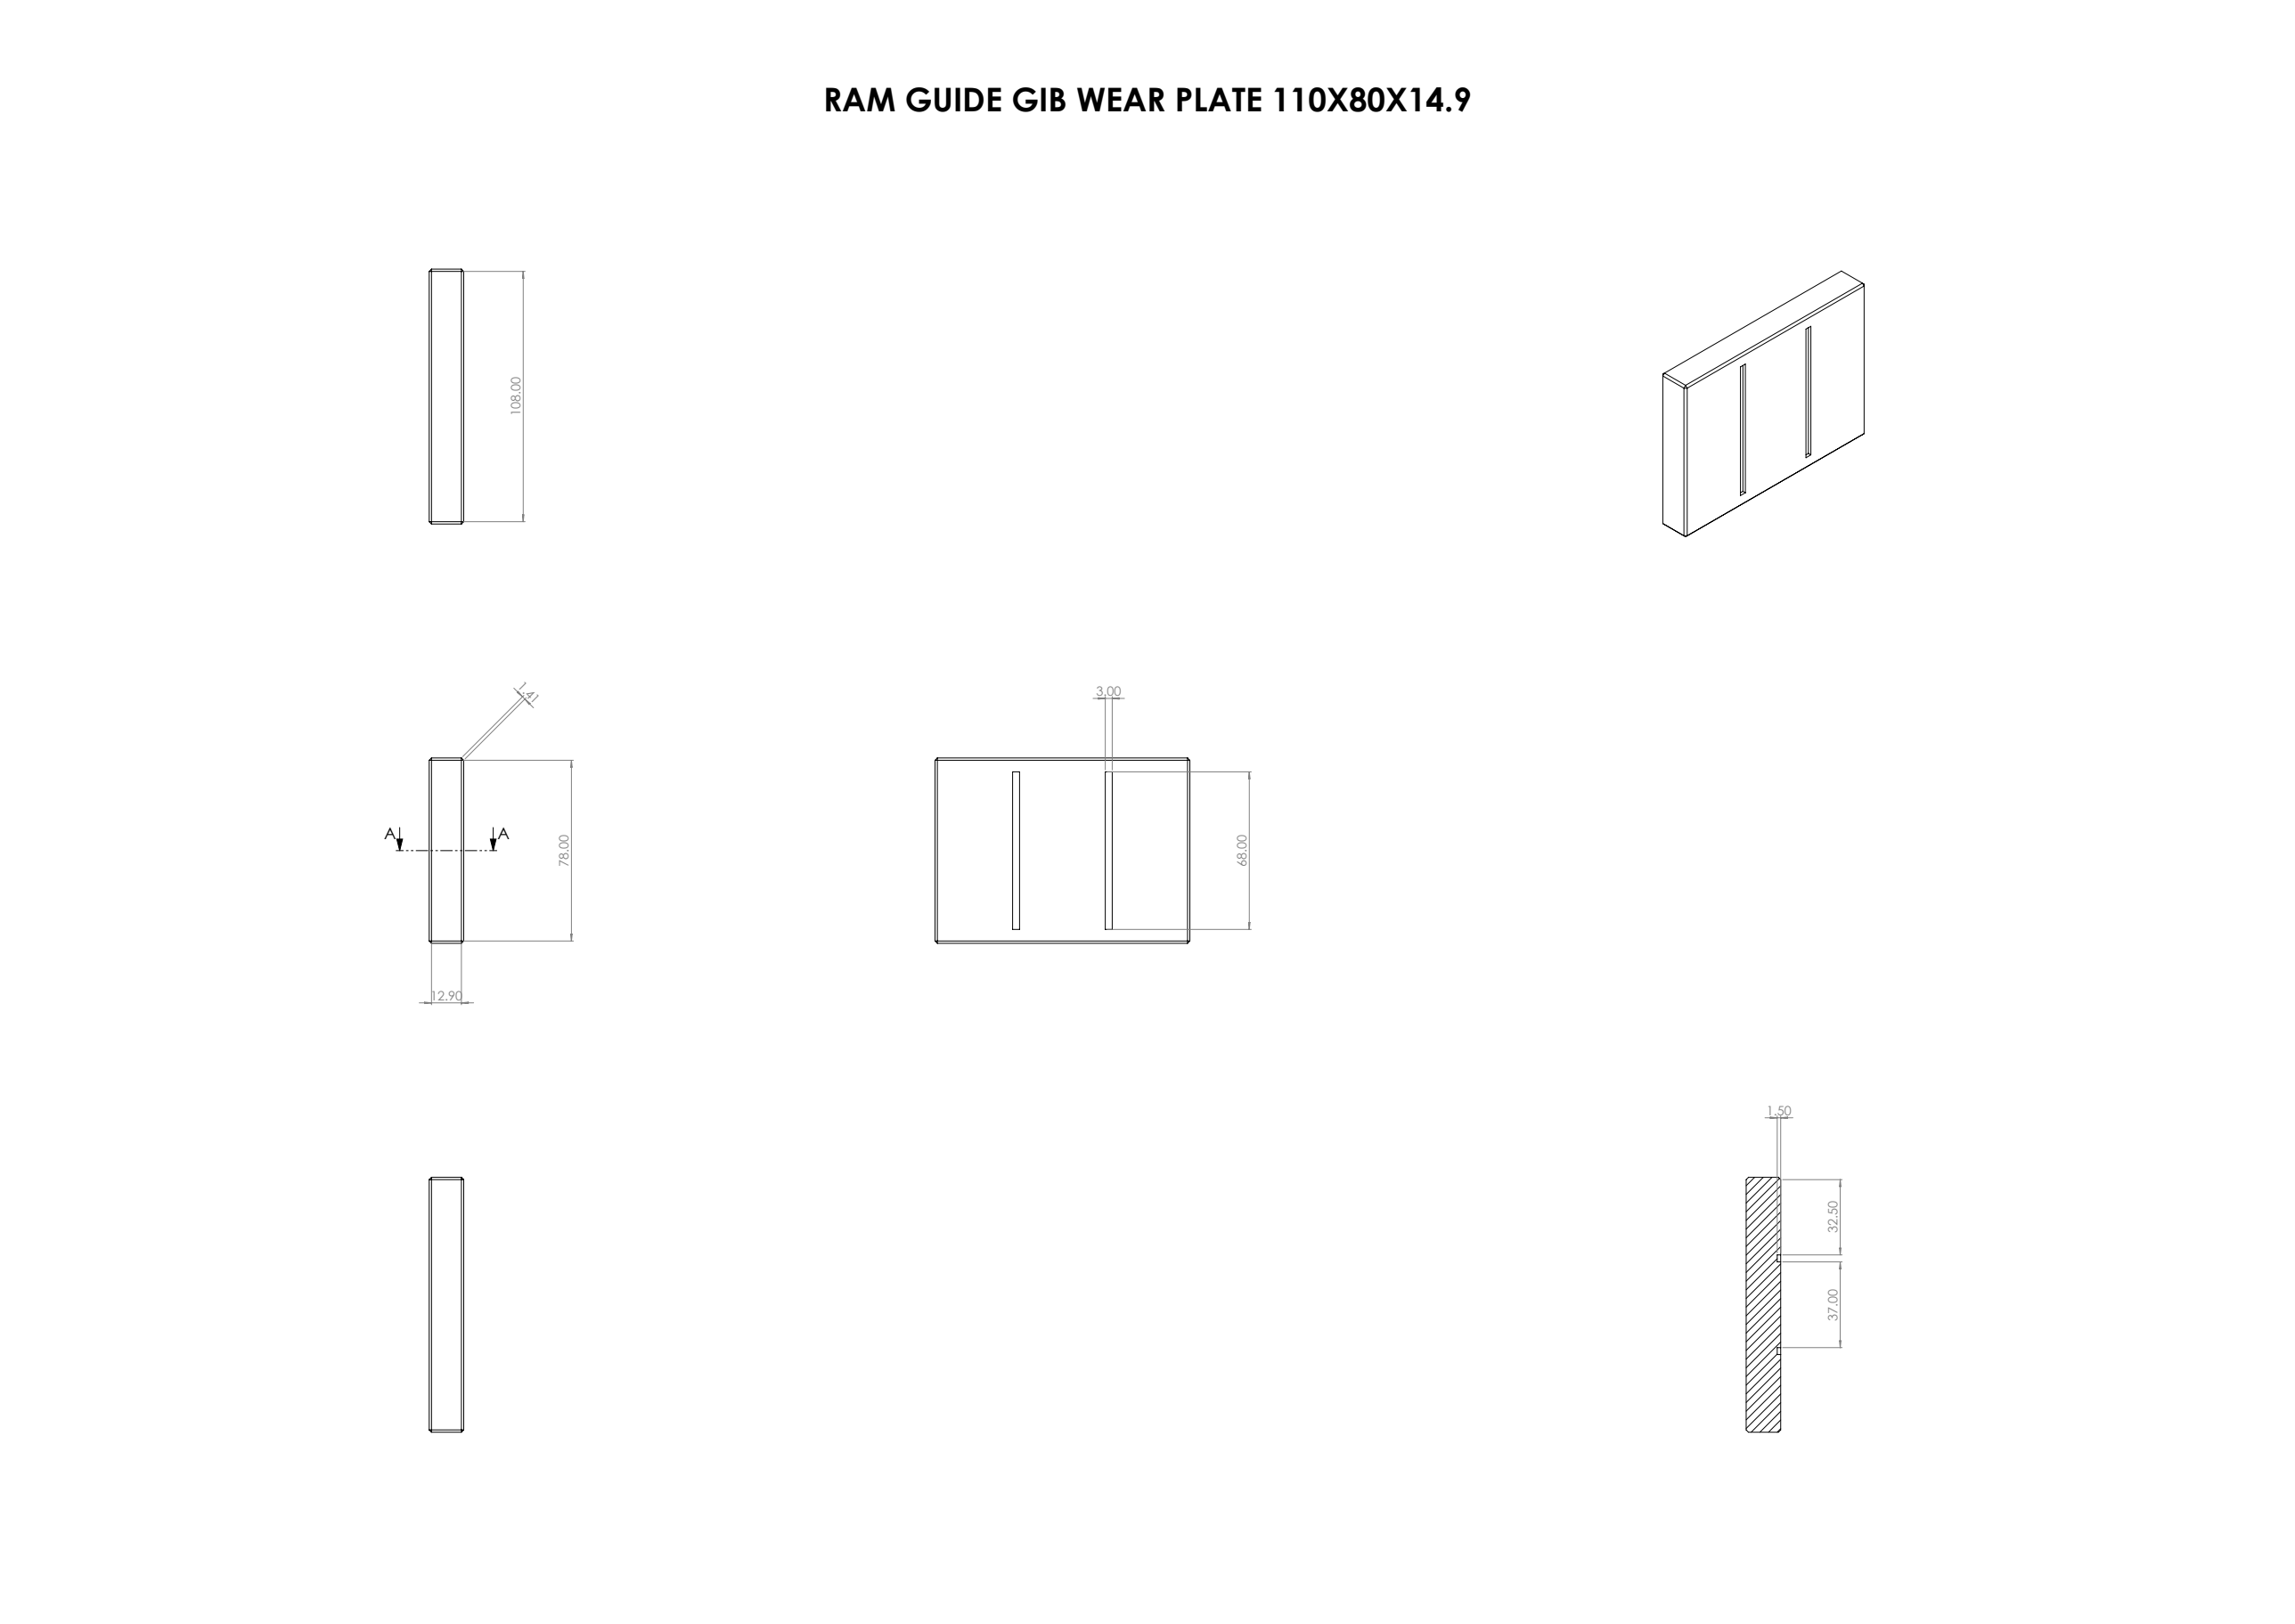
ISO-10303-21;
HEADER;
/* Generated by software containing ST-Developer
 * from STEP Tools, Inc. (www.steptools.com) 
 */

FILE_DESCRIPTION(
/* description */ (''),
/* implementation_level */ '2;1');

FILE_NAME(
/* name */ '10_Ram_Guide_Gib_Wear_Plate_110x80x14.9.step',
/* time_stamp */ '2026-10-19T23:58:09-07:00',
/* author */ (''),
/* organization */ (''),
/* preprocessor_version */ 'ST-DEVELOPER v20.2',
/* originating_system */ 'Autodesk Translation Framework v15.15.0.0',
/* authorisation */ '');

FILE_SCHEMA (('AP203_CONFIGURATION_CONTROLLED_3D_DESIGN_OF_MECHANICAL_PARTS_AND_ASSEMBLIES_MIM_LF { 1 0 10303 203 3 1 4 }',
'AUTOMOTIVE_DESIGN { 1 0 10303 214 3 1 1 }','INTEGRATED_CNC_SCHEMA','MODEL_BASED_INTEGRATED_MANUFACTURING_SCHEMA',
'PROCESS_PLANNING_SCHEMA','AP242_MANAGED_MODEL_BASED_3D_ENGINEERING_MIM_LF { 1 0 10303 442 3 1 4 }'));
ENDSEC;

DATA;
#10=MECHANICAL_DESIGN_GEOMETRIC_PRESENTATION_REPRESENTATION('',(#413),#70757);
#383=SHAPE_REPRESENTATION_RELATIONSHIP('SRR','None',#70824,#398);
#398=ADVANCED_BREP_SHAPE_REPRESENTATION('',(#473),#70748);
#413=STYLED_ITEM('',(#71040),#473);
#473=MANIFOLD_SOLID_BREP('Gib',#26878);
#862=FACE_BOUND('',#4417,.T.);
#863=FACE_BOUND('',#4418,.T.);
#1799=PLANE('',#27511);
#1800=PLANE('',#27512);
#1801=PLANE('',#27513);
#1802=PLANE('',#27514);
#1803=PLANE('',#27515);
#1804=PLANE('',#27516);
#1805=PLANE('',#27517);
#1806=PLANE('',#27518);
#1807=PLANE('',#27519);
#1808=PLANE('',#27520);
#1809=PLANE('',#27521);
#1810=PLANE('',#27522);
#1811=PLANE('',#27523);
#1812=PLANE('',#27524);
#1813=PLANE('',#27525);
#1814=PLANE('',#27526);
#1815=PLANE('',#27527);
#1816=PLANE('',#27528);
#1817=PLANE('',#27529);
#1818=PLANE('',#27530);
#1819=PLANE('',#27531);
#1820=PLANE('',#27532);
#1821=PLANE('',#27533);
#1822=PLANE('',#27534);
#1823=PLANE('',#27535);
#1824=PLANE('',#27536);
#1825=PLANE('',#27537);
#1826=PLANE('',#27538);
#1827=PLANE('',#27539);
#1828=PLANE('',#27540);
#1829=PLANE('',#27541);
#1830=PLANE('',#27542);
#1831=PLANE('',#27543);
#1832=PLANE('',#27544);
#1833=PLANE('',#27545);
#1834=PLANE('',#27546);
#2876=FACE_OUTER_BOUND('',#4382,.T.);
#2877=FACE_OUTER_BOUND('',#4383,.T.);
#2878=FACE_OUTER_BOUND('',#4384,.T.);
#2879=FACE_OUTER_BOUND('',#4385,.T.);
#2880=FACE_OUTER_BOUND('',#4386,.T.);
#2881=FACE_OUTER_BOUND('',#4387,.T.);
#2882=FACE_OUTER_BOUND('',#4388,.T.);
#2883=FACE_OUTER_BOUND('',#4389,.T.);
#2884=FACE_OUTER_BOUND('',#4390,.T.);
#2885=FACE_OUTER_BOUND('',#4391,.T.);
#2886=FACE_OUTER_BOUND('',#4392,.T.);
#2887=FACE_OUTER_BOUND('',#4393,.T.);
#2888=FACE_OUTER_BOUND('',#4394,.T.);
#2889=FACE_OUTER_BOUND('',#4395,.T.);
#2890=FACE_OUTER_BOUND('',#4396,.T.);
#2891=FACE_OUTER_BOUND('',#4397,.T.);
#2892=FACE_OUTER_BOUND('',#4398,.T.);
#2893=FACE_OUTER_BOUND('',#4399,.T.);
#2894=FACE_OUTER_BOUND('',#4400,.T.);
#2895=FACE_OUTER_BOUND('',#4401,.T.);
#2896=FACE_OUTER_BOUND('',#4402,.T.);
#2897=FACE_OUTER_BOUND('',#4403,.T.);
#2898=FACE_OUTER_BOUND('',#4404,.T.);
#2899=FACE_OUTER_BOUND('',#4405,.T.);
#2900=FACE_OUTER_BOUND('',#4406,.T.);
#2901=FACE_OUTER_BOUND('',#4407,.T.);
#2902=FACE_OUTER_BOUND('',#4408,.T.);
#2903=FACE_OUTER_BOUND('',#4409,.T.);
#2904=FACE_OUTER_BOUND('',#4410,.T.);
#2905=FACE_OUTER_BOUND('',#4411,.T.);
#2906=FACE_OUTER_BOUND('',#4412,.T.);
#2907=FACE_OUTER_BOUND('',#4413,.T.);
#2908=FACE_OUTER_BOUND('',#4414,.T.);
#2909=FACE_OUTER_BOUND('',#4415,.T.);
#2910=FACE_OUTER_BOUND('',#4416,.T.);
#2911=FACE_OUTER_BOUND('',#4419,.T.);
#4382=EDGE_LOOP('',(#19138,#19139,#19140,#19141));
#4383=EDGE_LOOP('',(#19142,#19143,#19144,#19145));
#4384=EDGE_LOOP('',(#19146,#19147,#19148,#19149));
#4385=EDGE_LOOP('',(#19150,#19151,#19152,#19153));
#4386=EDGE_LOOP('',(#19154,#19155,#19156,#19157));
#4387=EDGE_LOOP('',(#19158,#19159,#19160,#19161));
#4388=EDGE_LOOP('',(#19162,#19163,#19164,#19165));
#4389=EDGE_LOOP('',(#19166,#19167,#19168,#19169));
#4390=EDGE_LOOP('',(#19170,#19171,#19172,#19173));
#4391=EDGE_LOOP('',(#19174,#19175,#19176,#19177));
#4392=EDGE_LOOP('',(#19178,#19179,#19180));
#4393=EDGE_LOOP('',(#19181,#19182,#19183));
#4394=EDGE_LOOP('',(#19184,#19185,#19186));
#4395=EDGE_LOOP('',(#19187,#19188,#19189));
#4396=EDGE_LOOP('',(#19190,#19191,#19192));
#4397=EDGE_LOOP('',(#19193,#19194,#19195,#19196));
#4398=EDGE_LOOP('',(#19197,#19198,#19199));
#4399=EDGE_LOOP('',(#19200,#19201,#19202));
#4400=EDGE_LOOP('',(#19203,#19204,#19205,#19206));
#4401=EDGE_LOOP('',(#19207,#19208,#19209,#19210));
#4402=EDGE_LOOP('',(#19211,#19212,#19213));
#4403=EDGE_LOOP('',(#19214,#19215,#19216,#19217));
#4404=EDGE_LOOP('',(#19218,#19219,#19220,#19221));
#4405=EDGE_LOOP('',(#19222,#19223,#19224,#19225));
#4406=EDGE_LOOP('',(#19226,#19227,#19228,#19229));
#4407=EDGE_LOOP('',(#19230,#19231,#19232,#19233));
#4408=EDGE_LOOP('',(#19234,#19235,#19236,#19237));
#4409=EDGE_LOOP('',(#19238,#19239,#19240,#19241));
#4410=EDGE_LOOP('',(#19242,#19243,#19244,#19245));
#4411=EDGE_LOOP('',(#19246,#19247,#19248,#19249));
#4412=EDGE_LOOP('',(#19250,#19251,#19252,#19253));
#4413=EDGE_LOOP('',(#19254,#19255,#19256,#19257));
#4414=EDGE_LOOP('',(#19258,#19259,#19260,#19261));
#4415=EDGE_LOOP('',(#19262,#19263,#19264,#19265));
#4416=EDGE_LOOP('',(#19266,#19267,#19268,#19269));
#4417=EDGE_LOOP('',(#19270,#19271,#19272,#19273));
#4418=EDGE_LOOP('',(#19274,#19275,#19276,#19277));
#4419=EDGE_LOOP('',(#19278,#19279,#19280,#19281));
#5977=LINE('',#47443,#8474);
#5978=LINE('',#47445,#8475);
#5979=LINE('',#47447,#8476);
#5980=LINE('',#47448,#8477);
#5981=LINE('',#47451,#8478);
#5982=LINE('',#47453,#8479);
#5983=LINE('',#47454,#8480);
#5984=LINE('',#47457,#8481);
#5985=LINE('',#47459,#8482);
#5986=LINE('',#47460,#8483);
#5987=LINE('',#47462,#8484);
#5988=LINE('',#47463,#8485);
#5989=LINE('',#47468,#8486);
#5990=LINE('',#47470,#8487);
#5991=LINE('',#47472,#8488);
#5992=LINE('',#47473,#8489);
#5993=LINE('',#47476,#8490);
#5994=LINE('',#47478,#8491);
#5995=LINE('',#47479,#8492);
#5996=LINE('',#47482,#8493);
#5997=LINE('',#47484,#8494);
#5998=LINE('',#47485,#8495);
#5999=LINE('',#47487,#8496);
#6000=LINE('',#47488,#8497);
#6001=LINE('',#47493,#8498);
#6002=LINE('',#47495,#8499);
#6003=LINE('',#47496,#8500);
#6004=LINE('',#47500,#8501);
#6005=LINE('',#47502,#8502);
#6006=LINE('',#47503,#8503);
#6007=LINE('',#47507,#8504);
#6008=LINE('',#47509,#8505);
#6009=LINE('',#47510,#8506);
#6010=LINE('',#47514,#8507);
#6011=LINE('',#47516,#8508);
#6012=LINE('',#47517,#8509);
#6013=LINE('',#47521,#8510);
#6014=LINE('',#47523,#8511);
#6015=LINE('',#47524,#8512);
#6016=LINE('',#47526,#8513);
#6017=LINE('',#47527,#8514);
#6018=LINE('',#47531,#8515);
#6019=LINE('',#47533,#8516);
#6020=LINE('',#47534,#8517);
#6021=LINE('',#47538,#8518);
#6022=LINE('',#47540,#8519);
#6023=LINE('',#47541,#8520);
#6024=LINE('',#47543,#8521);
#6025=LINE('',#47544,#8522);
#6026=LINE('',#47546,#8523);
#6027=LINE('',#47547,#8524);
#6028=LINE('',#47551,#8525);
#6029=LINE('',#47553,#8526);
#6030=LINE('',#47554,#8527);
#6031=LINE('',#47556,#8528);
#6032=LINE('',#47557,#8529);
#6033=LINE('',#47559,#8530);
#6034=LINE('',#47560,#8531);
#6035=LINE('',#47562,#8532);
#6036=LINE('',#47563,#8533);
#6037=LINE('',#47565,#8534);
#6038=LINE('',#47566,#8535);
#6039=LINE('',#47568,#8536);
#6040=LINE('',#47569,#8537);
#6041=LINE('',#47571,#8538);
#6042=LINE('',#47572,#8539);
#6043=LINE('',#47574,#8540);
#6044=LINE('',#47575,#8541);
#6045=LINE('',#47577,#8542);
#6046=LINE('',#47578,#8543);
#6047=LINE('',#47580,#8544);
#6048=LINE('',#47581,#8545);
#8474=VECTOR('',#30250,1.);
#8475=VECTOR('',#30251,1.);
#8476=VECTOR('',#30252,1.);
#8477=VECTOR('',#30253,1.);
#8478=VECTOR('',#30256,1.);
#8479=VECTOR('',#30257,1.);
#8480=VECTOR('',#30258,1.);
#8481=VECTOR('',#30261,1.);
#8482=VECTOR('',#30262,1.);
#8483=VECTOR('',#30263,1.);
#8484=VECTOR('',#30266,1.);
#8485=VECTOR('',#30267,1.);
#8486=VECTOR('',#30272,1.);
#8487=VECTOR('',#30273,1.);
#8488=VECTOR('',#30274,1.);
#8489=VECTOR('',#30275,1.);
#8490=VECTOR('',#30278,1.);
#8491=VECTOR('',#30279,1.);
#8492=VECTOR('',#30280,1.);
#8493=VECTOR('',#30283,1.);
#8494=VECTOR('',#30284,1.);
#8495=VECTOR('',#30285,1.);
#8496=VECTOR('',#30288,1.);
#8497=VECTOR('',#30289,1.);
#8498=VECTOR('',#30294,1.);
#8499=VECTOR('',#30295,1.);
#8500=VECTOR('',#30296,1.);
#8501=VECTOR('',#30299,1.);
#8502=VECTOR('',#30300,1.);
#8503=VECTOR('',#30301,1.);
#8504=VECTOR('',#30304,1.);
#8505=VECTOR('',#30305,1.);
#8506=VECTOR('',#30306,1.);
#8507=VECTOR('',#30309,1.);
#8508=VECTOR('',#30310,1.);
#8509=VECTOR('',#30311,1.);
#8510=VECTOR('',#30314,1.);
#8511=VECTOR('',#30315,1.);
#8512=VECTOR('',#30316,1.);
#8513=VECTOR('',#30319,1.);
#8514=VECTOR('',#30320,1.);
#8515=VECTOR('',#30323,1.);
#8516=VECTOR('',#30324,1.);
#8517=VECTOR('',#30325,1.);
#8518=VECTOR('',#30328,1.);
#8519=VECTOR('',#30329,1.);
#8520=VECTOR('',#30330,1.);
#8521=VECTOR('',#30333,1.);
#8522=VECTOR('',#30334,1.);
#8523=VECTOR('',#30337,1.);
#8524=VECTOR('',#30338,1.);
#8525=VECTOR('',#30341,1.);
#8526=VECTOR('',#30342,1.);
#8527=VECTOR('',#30343,1.);
#8528=VECTOR('',#30346,1.);
#8529=VECTOR('',#30347,1.);
#8530=VECTOR('',#30350,1.);
#8531=VECTOR('',#30351,1.);
#8532=VECTOR('',#30354,1.);
#8533=VECTOR('',#30355,1.);
#8534=VECTOR('',#30358,1.);
#8535=VECTOR('',#30359,1.);
#8536=VECTOR('',#30362,1.);
#8537=VECTOR('',#30363,1.);
#8538=VECTOR('',#30366,1.);
#8539=VECTOR('',#30367,1.);
#8540=VECTOR('',#30370,1.);
#8541=VECTOR('',#30371,1.);
#8542=VECTOR('',#30374,1.);
#8543=VECTOR('',#30375,1.);
#8544=VECTOR('',#30378,1.);
#8545=VECTOR('',#30379,1.);
#11664=VERTEX_POINT('',#47441);
#11665=VERTEX_POINT('',#47442);
#11666=VERTEX_POINT('',#47444);
#11667=VERTEX_POINT('',#47446);
#11668=VERTEX_POINT('',#47450);
#11669=VERTEX_POINT('',#47452);
#11670=VERTEX_POINT('',#47456);
#11671=VERTEX_POINT('',#47458);
#11672=VERTEX_POINT('',#47466);
#11673=VERTEX_POINT('',#47467);
#11674=VERTEX_POINT('',#47469);
#11675=VERTEX_POINT('',#47471);
#11676=VERTEX_POINT('',#47475);
#11677=VERTEX_POINT('',#47477);
#11678=VERTEX_POINT('',#47481);
#11679=VERTEX_POINT('',#47483);
#11680=VERTEX_POINT('',#47491);
#11681=VERTEX_POINT('',#47492);
#11682=VERTEX_POINT('',#47494);
#11683=VERTEX_POINT('',#47498);
#11684=VERTEX_POINT('',#47499);
#11685=VERTEX_POINT('',#47501);
#11686=VERTEX_POINT('',#47505);
#11687=VERTEX_POINT('',#47506);
#11688=VERTEX_POINT('',#47508);
#11689=VERTEX_POINT('',#47512);
#11690=VERTEX_POINT('',#47513);
#11691=VERTEX_POINT('',#47515);
#11692=VERTEX_POINT('',#47519);
#11693=VERTEX_POINT('',#47520);
#11694=VERTEX_POINT('',#47522);
#11695=VERTEX_POINT('',#47529);
#11696=VERTEX_POINT('',#47530);
#11697=VERTEX_POINT('',#47532);
#11698=VERTEX_POINT('',#47536);
#11699=VERTEX_POINT('',#47537);
#11700=VERTEX_POINT('',#47539);
#11701=VERTEX_POINT('',#47549);
#11702=VERTEX_POINT('',#47550);
#11703=VERTEX_POINT('',#47552);
#14422=EDGE_CURVE('',#11664,#11665,#5977,.T.);
#14423=EDGE_CURVE('',#11664,#11666,#5978,.T.);
#14424=EDGE_CURVE('',#11666,#11667,#5979,.T.);
#14425=EDGE_CURVE('',#11665,#11667,#5980,.T.);
#14426=EDGE_CURVE('',#11668,#11664,#5981,.T.);
#14427=EDGE_CURVE('',#11668,#11669,#5982,.T.);
#14428=EDGE_CURVE('',#11669,#11666,#5983,.T.);
#14429=EDGE_CURVE('',#11670,#11668,#5984,.T.);
#14430=EDGE_CURVE('',#11670,#11671,#5985,.T.);
#14431=EDGE_CURVE('',#11671,#11669,#5986,.T.);
#14432=EDGE_CURVE('',#11665,#11670,#5987,.T.);
#14433=EDGE_CURVE('',#11667,#11671,#5988,.T.);
#14434=EDGE_CURVE('',#11672,#11673,#5989,.T.);
#14435=EDGE_CURVE('',#11672,#11674,#5990,.T.);
#14436=EDGE_CURVE('',#11674,#11675,#5991,.T.);
#14437=EDGE_CURVE('',#11673,#11675,#5992,.T.);
#14438=EDGE_CURVE('',#11676,#11672,#5993,.T.);
#14439=EDGE_CURVE('',#11676,#11677,#5994,.T.);
#14440=EDGE_CURVE('',#11677,#11674,#5995,.T.);
#14441=EDGE_CURVE('',#11678,#11676,#5996,.T.);
#14442=EDGE_CURVE('',#11678,#11679,#5997,.T.);
#14443=EDGE_CURVE('',#11679,#11677,#5998,.T.);
#14444=EDGE_CURVE('',#11673,#11678,#5999,.T.);
#14445=EDGE_CURVE('',#11675,#11679,#6000,.T.);
#14446=EDGE_CURVE('',#11680,#11681,#6001,.T.);
#14447=EDGE_CURVE('',#11682,#11680,#6002,.T.);
#14448=EDGE_CURVE('',#11681,#11682,#6003,.T.);
#14449=EDGE_CURVE('',#11683,#11684,#6004,.T.);
#14450=EDGE_CURVE('',#11685,#11683,#6005,.T.);
#14451=EDGE_CURVE('',#11684,#11685,#6006,.T.);
#14452=EDGE_CURVE('',#11686,#11687,#6007,.T.);
#14453=EDGE_CURVE('',#11688,#11686,#6008,.T.);
#14454=EDGE_CURVE('',#11687,#11688,#6009,.T.);
#14455=EDGE_CURVE('',#11689,#11690,#6010,.T.);
#14456=EDGE_CURVE('',#11691,#11689,#6011,.T.);
#14457=EDGE_CURVE('',#11690,#11691,#6012,.T.);
#14458=EDGE_CURVE('',#11692,#11693,#6013,.T.);
#14459=EDGE_CURVE('',#11694,#11692,#6014,.T.);
#14460=EDGE_CURVE('',#11693,#11694,#6015,.T.);
#14461=EDGE_CURVE('',#11692,#11687,#6016,.T.);
#14462=EDGE_CURVE('',#11688,#11694,#6017,.T.);
#14463=EDGE_CURVE('',#11695,#11696,#6018,.T.);
#14464=EDGE_CURVE('',#11697,#11695,#6019,.T.);
#14465=EDGE_CURVE('',#11696,#11697,#6020,.T.);
#14466=EDGE_CURVE('',#11698,#11699,#6021,.T.);
#14467=EDGE_CURVE('',#11700,#11698,#6022,.T.);
#14468=EDGE_CURVE('',#11699,#11700,#6023,.T.);
#14469=EDGE_CURVE('',#11686,#11700,#6024,.T.);
#14470=EDGE_CURVE('',#11698,#11688,#6025,.T.);
#14471=EDGE_CURVE('',#11689,#11699,#6026,.T.);
#14472=EDGE_CURVE('',#11700,#11691,#6027,.T.);
#14473=EDGE_CURVE('',#11701,#11702,#6028,.T.);
#14474=EDGE_CURVE('',#11703,#11701,#6029,.T.);
#14475=EDGE_CURVE('',#11702,#11703,#6030,.T.);
#14476=EDGE_CURVE('',#11701,#11693,#6031,.T.);
#14477=EDGE_CURVE('',#11694,#11703,#6032,.T.);
#14478=EDGE_CURVE('',#11699,#11702,#6033,.T.);
#14479=EDGE_CURVE('',#11703,#11698,#6034,.T.);
#14480=EDGE_CURVE('',#11695,#11701,#6035,.T.);
#14481=EDGE_CURVE('',#11702,#11697,#6036,.T.);
#14482=EDGE_CURVE('',#11690,#11696,#6037,.T.);
#14483=EDGE_CURVE('',#11697,#11689,#6038,.T.);
#14484=EDGE_CURVE('',#11696,#11684,#6039,.T.);
#14485=EDGE_CURVE('',#11685,#11695,#6040,.T.);
#14486=EDGE_CURVE('',#11683,#11692,#6041,.T.);
#14487=EDGE_CURVE('',#11693,#11685,#6042,.T.);
#14488=EDGE_CURVE('',#11681,#11690,#6043,.T.);
#14489=EDGE_CURVE('',#11691,#11680,#6044,.T.);
#14490=EDGE_CURVE('',#11680,#11686,#6045,.T.);
#14491=EDGE_CURVE('',#11687,#11682,#6046,.T.);
#14492=EDGE_CURVE('',#11684,#11681,#6047,.T.);
#14493=EDGE_CURVE('',#11682,#11683,#6048,.T.);
#19138=ORIENTED_EDGE('',*,*,#14422,.F.);
#19139=ORIENTED_EDGE('',*,*,#14423,.T.);
#19140=ORIENTED_EDGE('',*,*,#14424,.T.);
#19141=ORIENTED_EDGE('',*,*,#14425,.F.);
#19142=ORIENTED_EDGE('',*,*,#14426,.F.);
#19143=ORIENTED_EDGE('',*,*,#14427,.T.);
#19144=ORIENTED_EDGE('',*,*,#14428,.T.);
#19145=ORIENTED_EDGE('',*,*,#14423,.F.);
#19146=ORIENTED_EDGE('',*,*,#14429,.F.);
#19147=ORIENTED_EDGE('',*,*,#14430,.T.);
#19148=ORIENTED_EDGE('',*,*,#14431,.T.);
#19149=ORIENTED_EDGE('',*,*,#14427,.F.);
#19150=ORIENTED_EDGE('',*,*,#14432,.F.);
#19151=ORIENTED_EDGE('',*,*,#14425,.T.);
#19152=ORIENTED_EDGE('',*,*,#14433,.T.);
#19153=ORIENTED_EDGE('',*,*,#14430,.F.);
#19154=ORIENTED_EDGE('',*,*,#14433,.F.);
#19155=ORIENTED_EDGE('',*,*,#14424,.F.);
#19156=ORIENTED_EDGE('',*,*,#14428,.F.);
#19157=ORIENTED_EDGE('',*,*,#14431,.F.);
#19158=ORIENTED_EDGE('',*,*,#14434,.F.);
#19159=ORIENTED_EDGE('',*,*,#14435,.T.);
#19160=ORIENTED_EDGE('',*,*,#14436,.T.);
#19161=ORIENTED_EDGE('',*,*,#14437,.F.);
#19162=ORIENTED_EDGE('',*,*,#14438,.F.);
#19163=ORIENTED_EDGE('',*,*,#14439,.T.);
#19164=ORIENTED_EDGE('',*,*,#14440,.T.);
#19165=ORIENTED_EDGE('',*,*,#14435,.F.);
#19166=ORIENTED_EDGE('',*,*,#14441,.F.);
#19167=ORIENTED_EDGE('',*,*,#14442,.T.);
#19168=ORIENTED_EDGE('',*,*,#14443,.T.);
#19169=ORIENTED_EDGE('',*,*,#14439,.F.);
#19170=ORIENTED_EDGE('',*,*,#14444,.F.);
#19171=ORIENTED_EDGE('',*,*,#14437,.T.);
#19172=ORIENTED_EDGE('',*,*,#14445,.T.);
#19173=ORIENTED_EDGE('',*,*,#14442,.F.);
#19174=ORIENTED_EDGE('',*,*,#14445,.F.);
#19175=ORIENTED_EDGE('',*,*,#14436,.F.);
#19176=ORIENTED_EDGE('',*,*,#14440,.F.);
#19177=ORIENTED_EDGE('',*,*,#14443,.F.);
#19178=ORIENTED_EDGE('',*,*,#14446,.F.);
#19179=ORIENTED_EDGE('',*,*,#14447,.F.);
#19180=ORIENTED_EDGE('',*,*,#14448,.F.);
#19181=ORIENTED_EDGE('',*,*,#14449,.F.);
#19182=ORIENTED_EDGE('',*,*,#14450,.F.);
#19183=ORIENTED_EDGE('',*,*,#14451,.F.);
#19184=ORIENTED_EDGE('',*,*,#14452,.F.);
#19185=ORIENTED_EDGE('',*,*,#14453,.F.);
#19186=ORIENTED_EDGE('',*,*,#14454,.F.);
#19187=ORIENTED_EDGE('',*,*,#14455,.F.);
#19188=ORIENTED_EDGE('',*,*,#14456,.F.);
#19189=ORIENTED_EDGE('',*,*,#14457,.F.);
#19190=ORIENTED_EDGE('',*,*,#14458,.F.);
#19191=ORIENTED_EDGE('',*,*,#14459,.F.);
#19192=ORIENTED_EDGE('',*,*,#14460,.F.);
#19193=ORIENTED_EDGE('',*,*,#14459,.T.);
#19194=ORIENTED_EDGE('',*,*,#14461,.T.);
#19195=ORIENTED_EDGE('',*,*,#14454,.T.);
#19196=ORIENTED_EDGE('',*,*,#14462,.T.);
#19197=ORIENTED_EDGE('',*,*,#14463,.F.);
#19198=ORIENTED_EDGE('',*,*,#14464,.F.);
#19199=ORIENTED_EDGE('',*,*,#14465,.F.);
#19200=ORIENTED_EDGE('',*,*,#14466,.F.);
#19201=ORIENTED_EDGE('',*,*,#14467,.F.);
#19202=ORIENTED_EDGE('',*,*,#14468,.F.);
#19203=ORIENTED_EDGE('',*,*,#14453,.T.);
#19204=ORIENTED_EDGE('',*,*,#14469,.T.);
#19205=ORIENTED_EDGE('',*,*,#14467,.T.);
#19206=ORIENTED_EDGE('',*,*,#14470,.T.);
#19207=ORIENTED_EDGE('',*,*,#14456,.T.);
#19208=ORIENTED_EDGE('',*,*,#14471,.T.);
#19209=ORIENTED_EDGE('',*,*,#14468,.T.);
#19210=ORIENTED_EDGE('',*,*,#14472,.T.);
#19211=ORIENTED_EDGE('',*,*,#14473,.F.);
#19212=ORIENTED_EDGE('',*,*,#14474,.F.);
#19213=ORIENTED_EDGE('',*,*,#14475,.F.);
#19214=ORIENTED_EDGE('',*,*,#14474,.T.);
#19215=ORIENTED_EDGE('',*,*,#14476,.T.);
#19216=ORIENTED_EDGE('',*,*,#14460,.T.);
#19217=ORIENTED_EDGE('',*,*,#14477,.T.);
#19218=ORIENTED_EDGE('',*,*,#14466,.T.);
#19219=ORIENTED_EDGE('',*,*,#14478,.T.);
#19220=ORIENTED_EDGE('',*,*,#14475,.T.);
#19221=ORIENTED_EDGE('',*,*,#14479,.T.);
#19222=ORIENTED_EDGE('',*,*,#14464,.T.);
#19223=ORIENTED_EDGE('',*,*,#14480,.T.);
#19224=ORIENTED_EDGE('',*,*,#14473,.T.);
#19225=ORIENTED_EDGE('',*,*,#14481,.T.);
#19226=ORIENTED_EDGE('',*,*,#14455,.T.);
#19227=ORIENTED_EDGE('',*,*,#14482,.T.);
#19228=ORIENTED_EDGE('',*,*,#14465,.T.);
#19229=ORIENTED_EDGE('',*,*,#14483,.T.);
#19230=ORIENTED_EDGE('',*,*,#14463,.T.);
#19231=ORIENTED_EDGE('',*,*,#14484,.T.);
#19232=ORIENTED_EDGE('',*,*,#14451,.T.);
#19233=ORIENTED_EDGE('',*,*,#14485,.T.);
#19234=ORIENTED_EDGE('',*,*,#14450,.T.);
#19235=ORIENTED_EDGE('',*,*,#14486,.T.);
#19236=ORIENTED_EDGE('',*,*,#14458,.T.);
#19237=ORIENTED_EDGE('',*,*,#14487,.T.);
#19238=ORIENTED_EDGE('',*,*,#14446,.T.);
#19239=ORIENTED_EDGE('',*,*,#14488,.T.);
#19240=ORIENTED_EDGE('',*,*,#14457,.T.);
#19241=ORIENTED_EDGE('',*,*,#14489,.T.);
#19242=ORIENTED_EDGE('',*,*,#14447,.T.);
#19243=ORIENTED_EDGE('',*,*,#14490,.T.);
#19244=ORIENTED_EDGE('',*,*,#14452,.T.);
#19245=ORIENTED_EDGE('',*,*,#14491,.T.);
#19246=ORIENTED_EDGE('',*,*,#14449,.T.);
#19247=ORIENTED_EDGE('',*,*,#14492,.T.);
#19248=ORIENTED_EDGE('',*,*,#14448,.T.);
#19249=ORIENTED_EDGE('',*,*,#14493,.T.);
#19250=ORIENTED_EDGE('',*,*,#14461,.F.);
#19251=ORIENTED_EDGE('',*,*,#14486,.F.);
#19252=ORIENTED_EDGE('',*,*,#14493,.F.);
#19253=ORIENTED_EDGE('',*,*,#14491,.F.);
#19254=ORIENTED_EDGE('',*,*,#14462,.F.);
#19255=ORIENTED_EDGE('',*,*,#14470,.F.);
#19256=ORIENTED_EDGE('',*,*,#14479,.F.);
#19257=ORIENTED_EDGE('',*,*,#14477,.F.);
#19258=ORIENTED_EDGE('',*,*,#14469,.F.);
#19259=ORIENTED_EDGE('',*,*,#14490,.F.);
#19260=ORIENTED_EDGE('',*,*,#14489,.F.);
#19261=ORIENTED_EDGE('',*,*,#14472,.F.);
#19262=ORIENTED_EDGE('',*,*,#14471,.F.);
#19263=ORIENTED_EDGE('',*,*,#14483,.F.);
#19264=ORIENTED_EDGE('',*,*,#14481,.F.);
#19265=ORIENTED_EDGE('',*,*,#14478,.F.);
#19266=ORIENTED_EDGE('',*,*,#14476,.F.);
#19267=ORIENTED_EDGE('',*,*,#14480,.F.);
#19268=ORIENTED_EDGE('',*,*,#14485,.F.);
#19269=ORIENTED_EDGE('',*,*,#14487,.F.);
#19270=ORIENTED_EDGE('',*,*,#14422,.T.);
#19271=ORIENTED_EDGE('',*,*,#14432,.T.);
#19272=ORIENTED_EDGE('',*,*,#14429,.T.);
#19273=ORIENTED_EDGE('',*,*,#14426,.T.);
#19274=ORIENTED_EDGE('',*,*,#14434,.T.);
#19275=ORIENTED_EDGE('',*,*,#14444,.T.);
#19276=ORIENTED_EDGE('',*,*,#14441,.T.);
#19277=ORIENTED_EDGE('',*,*,#14438,.T.);
#19278=ORIENTED_EDGE('',*,*,#14482,.F.);
#19279=ORIENTED_EDGE('',*,*,#14488,.F.);
#19280=ORIENTED_EDGE('',*,*,#14492,.F.);
#19281=ORIENTED_EDGE('',*,*,#14484,.F.);
#25689=ADVANCED_FACE('',(#2876),#1799,.F.);
#25690=ADVANCED_FACE('',(#2877),#1800,.F.);
#25691=ADVANCED_FACE('',(#2878),#1801,.F.);
#25692=ADVANCED_FACE('',(#2879),#1802,.F.);
#25693=ADVANCED_FACE('',(#2880),#1803,.F.);
#25694=ADVANCED_FACE('',(#2881),#1804,.F.);
#25695=ADVANCED_FACE('',(#2882),#1805,.F.);
#25696=ADVANCED_FACE('',(#2883),#1806,.F.);
#25697=ADVANCED_FACE('',(#2884),#1807,.F.);
#25698=ADVANCED_FACE('',(#2885),#1808,.F.);
#25699=ADVANCED_FACE('',(#2886),#1809,.T.);
#25700=ADVANCED_FACE('',(#2887),#1810,.T.);
#25701=ADVANCED_FACE('',(#2888),#1811,.T.);
#25702=ADVANCED_FACE('',(#2889),#1812,.T.);
#25703=ADVANCED_FACE('',(#2890),#1813,.T.);
#25704=ADVANCED_FACE('',(#2891),#1814,.T.);
#25705=ADVANCED_FACE('',(#2892),#1815,.T.);
#25706=ADVANCED_FACE('',(#2893),#1816,.T.);
#25707=ADVANCED_FACE('',(#2894),#1817,.T.);
#25708=ADVANCED_FACE('',(#2895),#1818,.T.);
#25709=ADVANCED_FACE('',(#2896),#1819,.T.);
#25710=ADVANCED_FACE('',(#2897),#1820,.T.);
#25711=ADVANCED_FACE('',(#2898),#1821,.T.);
#25712=ADVANCED_FACE('',(#2899),#1822,.T.);
#25713=ADVANCED_FACE('',(#2900),#1823,.T.);
#25714=ADVANCED_FACE('',(#2901),#1824,.T.);
#25715=ADVANCED_FACE('',(#2902),#1825,.T.);
#25716=ADVANCED_FACE('',(#2903),#1826,.T.);
#25717=ADVANCED_FACE('',(#2904),#1827,.T.);
#25718=ADVANCED_FACE('',(#2905),#1828,.T.);
#25719=ADVANCED_FACE('',(#2906),#1829,.T.);
#25720=ADVANCED_FACE('',(#2907),#1830,.F.);
#25721=ADVANCED_FACE('',(#2908),#1831,.T.);
#25722=ADVANCED_FACE('',(#2909),#1832,.T.);
#25723=ADVANCED_FACE('',(#2910,#862,#863),#1833,.T.);
#25724=ADVANCED_FACE('',(#2911),#1834,.T.);
#26878=CLOSED_SHELL('',(#25689,#25690,#25691,#25692,#25693,#25694,#25695,
#25696,#25697,#25698,#25699,#25700,#25701,#25702,#25703,#25704,#25705,#25706,
#25707,#25708,#25709,#25710,#25711,#25712,#25713,#25714,#25715,#25716,#25717,
#25718,#25719,#25720,#25721,#25722,#25723,#25724));
#27510=AXIS2_PLACEMENT_3D('',#47439,#30246,#30247);
#27511=AXIS2_PLACEMENT_3D('',#47440,#30248,#30249);
#27512=AXIS2_PLACEMENT_3D('',#47449,#30254,#30255);
#27513=AXIS2_PLACEMENT_3D('',#47455,#30259,#30260);
#27514=AXIS2_PLACEMENT_3D('',#47461,#30264,#30265);
#27515=AXIS2_PLACEMENT_3D('',#47464,#30268,#30269);
#27516=AXIS2_PLACEMENT_3D('',#47465,#30270,#30271);
#27517=AXIS2_PLACEMENT_3D('',#47474,#30276,#30277);
#27518=AXIS2_PLACEMENT_3D('',#47480,#30281,#30282);
#27519=AXIS2_PLACEMENT_3D('',#47486,#30286,#30287);
#27520=AXIS2_PLACEMENT_3D('',#47489,#30290,#30291);
#27521=AXIS2_PLACEMENT_3D('',#47490,#30292,#30293);
#27522=AXIS2_PLACEMENT_3D('',#47497,#30297,#30298);
#27523=AXIS2_PLACEMENT_3D('',#47504,#30302,#30303);
#27524=AXIS2_PLACEMENT_3D('',#47511,#30307,#30308);
#27525=AXIS2_PLACEMENT_3D('',#47518,#30312,#30313);
#27526=AXIS2_PLACEMENT_3D('',#47525,#30317,#30318);
#27527=AXIS2_PLACEMENT_3D('',#47528,#30321,#30322);
#27528=AXIS2_PLACEMENT_3D('',#47535,#30326,#30327);
#27529=AXIS2_PLACEMENT_3D('',#47542,#30331,#30332);
#27530=AXIS2_PLACEMENT_3D('',#47545,#30335,#30336);
#27531=AXIS2_PLACEMENT_3D('',#47548,#30339,#30340);
#27532=AXIS2_PLACEMENT_3D('',#47555,#30344,#30345);
#27533=AXIS2_PLACEMENT_3D('',#47558,#30348,#30349);
#27534=AXIS2_PLACEMENT_3D('',#47561,#30352,#30353);
#27535=AXIS2_PLACEMENT_3D('',#47564,#30356,#30357);
#27536=AXIS2_PLACEMENT_3D('',#47567,#30360,#30361);
#27537=AXIS2_PLACEMENT_3D('',#47570,#30364,#30365);
#27538=AXIS2_PLACEMENT_3D('',#47573,#30368,#30369);
#27539=AXIS2_PLACEMENT_3D('',#47576,#30372,#30373);
#27540=AXIS2_PLACEMENT_3D('',#47579,#30376,#30377);
#27541=AXIS2_PLACEMENT_3D('',#47582,#30380,#30381);
#27542=AXIS2_PLACEMENT_3D('',#47583,#30382,#30383);
#27543=AXIS2_PLACEMENT_3D('',#47584,#30384,#30385);
#27544=AXIS2_PLACEMENT_3D('',#47585,#30386,#30387);
#27545=AXIS2_PLACEMENT_3D('',#47586,#30388,#30389);
#27546=AXIS2_PLACEMENT_3D('',#47587,#30390,#30391);
#30246=DIRECTION('axis',(0.,0.,1.));
#30247=DIRECTION('refdir',(1.,0.,0.));
#30248=DIRECTION('center_axis',(0.,0.,-1.));
#30249=DIRECTION('ref_axis',(0.,-1.,0.));
#30250=DIRECTION('',(0.,-1.,0.));
#30251=DIRECTION('',(-1.,0.,0.));
#30252=DIRECTION('',(0.,-1.,0.));
#30253=DIRECTION('',(-1.,0.,0.));
#30254=DIRECTION('center_axis',(0.,1.,0.));
#30255=DIRECTION('ref_axis',(0.,0.,-1.));
#30256=DIRECTION('',(0.,0.,-1.));
#30257=DIRECTION('',(-1.,0.,0.));
#30258=DIRECTION('',(0.,0.,-1.));
#30259=DIRECTION('center_axis',(0.,0.,1.));
#30260=DIRECTION('ref_axis',(0.,1.,0.));
#30261=DIRECTION('',(0.,1.,0.));
#30262=DIRECTION('',(-1.,0.,0.));
#30263=DIRECTION('',(0.,1.,0.));
#30264=DIRECTION('center_axis',(0.,-1.,0.));
#30265=DIRECTION('ref_axis',(0.,0.,1.));
#30266=DIRECTION('',(0.,0.,1.));
#30267=DIRECTION('',(0.,0.,1.));
#30268=DIRECTION('center_axis',(-1.,0.,0.));
#30269=DIRECTION('ref_axis',(0.,0.,1.));
#30270=DIRECTION('center_axis',(0.,0.,-1.));
#30271=DIRECTION('ref_axis',(0.,-1.,0.));
#30272=DIRECTION('',(0.,-1.,0.));
#30273=DIRECTION('',(-1.,0.,0.));
#30274=DIRECTION('',(0.,-1.,0.));
#30275=DIRECTION('',(-1.,0.,0.));
#30276=DIRECTION('center_axis',(0.,1.,0.));
#30277=DIRECTION('ref_axis',(0.,0.,-1.));
#30278=DIRECTION('',(0.,0.,-1.));
#30279=DIRECTION('',(-1.,0.,0.));
#30280=DIRECTION('',(0.,0.,-1.));
#30281=DIRECTION('center_axis',(0.,0.,1.));
#30282=DIRECTION('ref_axis',(0.,1.,0.));
#30283=DIRECTION('',(0.,1.,0.));
#30284=DIRECTION('',(-1.,0.,0.));
#30285=DIRECTION('',(0.,1.,0.));
#30286=DIRECTION('center_axis',(0.,-1.,0.));
#30287=DIRECTION('ref_axis',(0.,0.,1.));
#30288=DIRECTION('',(0.,0.,1.));
#30289=DIRECTION('',(0.,0.,1.));
#30290=DIRECTION('center_axis',(-1.,0.,0.));
#30291=DIRECTION('ref_axis',(0.,0.,1.));
#30292=DIRECTION('center_axis',(-0.577350269189615,-0.577350269189615,0.577350269189648));
#30293=DIRECTION('ref_axis',(0.707106781186568,0.,0.707106781186527));
#30294=DIRECTION('',(0.707106781186566,0.,0.707106781186529));
#30295=DIRECTION('',(-0.707106781186548,0.707106781186548,0.));
#30296=DIRECTION('',(0.,-0.707106781186568,-0.707106781186527));
#30297=DIRECTION('center_axis',(0.577350269189615,-0.577350269189615,0.577350269189648));
#30298=DIRECTION('ref_axis',(0.707106781186568,0.,-0.707106781186527));
#30299=DIRECTION('',(0.,0.707106781186568,0.707106781186527));
#30300=DIRECTION('',(-0.707106781186548,-0.707106781186548,0.));
#30301=DIRECTION('',(0.707106781186566,-3.14018491736764E-15,-0.707106781186529));
#30302=DIRECTION('center_axis',(-0.577350269189615,-0.577350269189612,-0.577350269189651));
#30303=DIRECTION('ref_axis',(-0.70710678118657,0.,0.707106781186525));
#30304=DIRECTION('',(0.707106781186548,-0.707106781186548,0.));
#30305=DIRECTION('',(-0.70710678118657,0.,0.707106781186526));
#30306=DIRECTION('',(6.28036983473528E-15,0.707106781186568,-0.707106781186527));
#30307=DIRECTION('center_axis',(-0.577350269189615,0.577350269189615,0.577350269189648));
#30308=DIRECTION('ref_axis',(0.707106781186568,0.,0.707106781186527));
#30309=DIRECTION('',(0.,-0.707106781186568,0.707106781186527));
#30310=DIRECTION('',(0.707106781186548,0.707106781186548,0.));
#30311=DIRECTION('',(-0.707106781186566,3.14018491736764E-15,-0.707106781186529));
#30312=DIRECTION('center_axis',(0.577350269189613,-0.577350269189613,-0.577350269189651));
#30313=DIRECTION('ref_axis',(-0.707106781186571,0.,-0.707106781186524));
#30314=DIRECTION('',(0.707106781186548,0.707106781186548,0.));
#30315=DIRECTION('',(6.28036983473528E-15,-0.707106781186568,0.707106781186527));
#30316=DIRECTION('',(-0.70710678118657,3.14018491736763E-15,-0.707106781186526));
#30317=DIRECTION('center_axis',(0.,-0.707106781186527,-0.707106781186568));
#30318=DIRECTION('ref_axis',(-1.,0.,0.));
#30319=DIRECTION('',(-1.,0.,0.));
#30320=DIRECTION('',(1.,0.,0.));
#30321=DIRECTION('center_axis',(0.577350269189615,0.577350269189615,0.577350269189648));
#30322=DIRECTION('ref_axis',(0.707106781186568,0.,-0.707106781186527));
#30323=DIRECTION('',(-0.707106781186566,0.,0.707106781186529));
#30324=DIRECTION('',(0.707106781186548,-0.707106781186548,0.));
#30325=DIRECTION('',(0.,0.707106781186568,-0.707106781186527));
#30326=DIRECTION('center_axis',(-0.577350269189613,0.577350269189613,-0.577350269189651));
#30327=DIRECTION('ref_axis',(-0.707106781186571,0.,0.707106781186524));
#30328=DIRECTION('',(-6.28036983473528E-15,0.707106781186568,0.707106781186527));
#30329=DIRECTION('',(0.70710678118657,-3.14018491736763E-15,-0.707106781186526));
#30330=DIRECTION('',(-0.707106781186548,-0.707106781186548,0.));
#30331=DIRECTION('center_axis',(-0.707106781186526,0.,-0.70710678118657));
#30332=DIRECTION('ref_axis',(-0.70710678118657,0.,0.707106781186526));
#30333=DIRECTION('',(0.,1.,0.));
#30334=DIRECTION('',(0.,-1.,0.));
#30335=DIRECTION('center_axis',(-0.707106781186548,0.707106781186548,0.));
#30336=DIRECTION('ref_axis',(0.,0.,1.));
#30337=DIRECTION('',(0.,0.,-1.));
#30338=DIRECTION('',(0.,0.,1.));
#30339=DIRECTION('center_axis',(0.577350269189615,0.577350269189612,-0.577350269189651));
#30340=DIRECTION('ref_axis',(-0.70710678118657,0.,-0.707106781186525));
#30341=DIRECTION('',(-0.707106781186548,0.707106781186548,0.));
#30342=DIRECTION('',(0.70710678118657,0.,0.707106781186526));
#30343=DIRECTION('',(-6.28036983473528E-15,-0.707106781186568,-0.707106781186527));
#30344=DIRECTION('center_axis',(0.707106781186526,0.,-0.70710678118657));
#30345=DIRECTION('ref_axis',(-0.70710678118657,0.,-0.707106781186526));
#30346=DIRECTION('',(0.,-1.,0.));
#30347=DIRECTION('',(0.,1.,0.));
#30348=DIRECTION('center_axis',(0.,0.707106781186527,-0.707106781186568));
#30349=DIRECTION('ref_axis',(-1.,0.,0.));
#30350=DIRECTION('',(1.,0.,0.));
#30351=DIRECTION('',(-1.,0.,0.));
#30352=DIRECTION('center_axis',(0.707106781186548,0.707106781186548,0.));
#30353=DIRECTION('ref_axis',(0.,0.,-1.));
#30354=DIRECTION('',(0.,0.,-1.));
#30355=DIRECTION('',(0.,0.,1.));
#30356=DIRECTION('center_axis',(0.,0.707106781186527,0.707106781186568));
#30357=DIRECTION('ref_axis',(1.,0.,0.));
#30358=DIRECTION('',(1.,0.,0.));
#30359=DIRECTION('',(-1.,0.,0.));
#30360=DIRECTION('center_axis',(0.707106781186529,0.,0.707106781186566));
#30361=DIRECTION('ref_axis',(0.707106781186566,0.,-0.707106781186529));
#30362=DIRECTION('',(0.,-1.,0.));
#30363=DIRECTION('',(0.,1.,0.));
#30364=DIRECTION('center_axis',(0.707106781186548,-0.707106781186548,0.));
#30365=DIRECTION('ref_axis',(0.,0.,-1.));
#30366=DIRECTION('',(0.,0.,-1.));
#30367=DIRECTION('',(0.,0.,1.));
#30368=DIRECTION('center_axis',(-0.707106781186529,0.,0.707106781186566));
#30369=DIRECTION('ref_axis',(0.707106781186566,0.,0.707106781186529));
#30370=DIRECTION('',(0.,1.,0.));
#30371=DIRECTION('',(0.,-1.,0.));
#30372=DIRECTION('center_axis',(-0.707106781186548,-0.707106781186548,0.));
#30373=DIRECTION('ref_axis',(0.,0.,1.));
#30374=DIRECTION('',(0.,0.,-1.));
#30375=DIRECTION('',(0.,0.,1.));
#30376=DIRECTION('center_axis',(0.,-0.707106781186527,0.707106781186568));
#30377=DIRECTION('ref_axis',(1.,0.,0.));
#30378=DIRECTION('',(-1.,0.,0.));
#30379=DIRECTION('',(1.,0.,0.));
#30380=DIRECTION('center_axis',(0.,-1.,0.));
#30381=DIRECTION('ref_axis',(1.,0.,0.));
#30382=DIRECTION('center_axis',(0.,0.,1.));
#30383=DIRECTION('ref_axis',(1.,0.,0.));
#30384=DIRECTION('center_axis',(-1.,0.,0.));
#30385=DIRECTION('ref_axis',(0.,-1.,0.));
#30386=DIRECTION('center_axis',(0.,1.,0.));
#30387=DIRECTION('ref_axis',(-1.,0.,0.));
#30388=DIRECTION('center_axis',(1.,0.,0.));
#30389=DIRECTION('ref_axis',(0.,1.,0.));
#30390=DIRECTION('center_axis',(0.,0.,1.));
#30391=DIRECTION('ref_axis',(1.,0.,0.));
#47439=CARTESIAN_POINT('',(0.,0.,0.));
#47440=CARTESIAN_POINT('Origin',(-4.505,3.4,68.85));
#47441=CARTESIAN_POINT('',(-4.505,3.4,68.85));
#47442=CARTESIAN_POINT('',(-4.505,-3.4,68.85));
#47443=CARTESIAN_POINT('',(-4.505,-0.3,68.85));
#47444=CARTESIAN_POINT('',(-4.655,3.4,68.85));
#47445=CARTESIAN_POINT('',(-4.505,3.4,68.85));
#47446=CARTESIAN_POINT('',(-4.655,-3.4,68.85));
#47447=CARTESIAN_POINT('',(-4.655,-3.4,68.85));
#47448=CARTESIAN_POINT('',(-4.505,-3.4,68.85));
#47449=CARTESIAN_POINT('Origin',(-4.505,3.4,69.15));
#47450=CARTESIAN_POINT('',(-4.505,3.4,69.15));
#47451=CARTESIAN_POINT('',(-4.505,3.4,67.325));
#47452=CARTESIAN_POINT('',(-4.655,3.4,69.15));
#47453=CARTESIAN_POINT('',(-4.505,3.4,69.15));
#47454=CARTESIAN_POINT('',(-4.655,3.4,68.85));
#47455=CARTESIAN_POINT('Origin',(-4.505,-3.4,69.15));
#47456=CARTESIAN_POINT('',(-4.505,-3.4,69.15));
#47457=CARTESIAN_POINT('',(-4.505,-3.7,69.15));
#47458=CARTESIAN_POINT('',(-4.655,-3.4,69.15));
#47459=CARTESIAN_POINT('',(-4.505,-3.4,69.15));
#47460=CARTESIAN_POINT('',(-4.655,3.4,69.15));
#47461=CARTESIAN_POINT('Origin',(-4.505,-3.4,68.85));
#47462=CARTESIAN_POINT('',(-4.505,-3.4,67.175));
#47463=CARTESIAN_POINT('',(-4.655,-3.4,69.15));
#47464=CARTESIAN_POINT('Origin',(-4.655,0.,69.));
#47465=CARTESIAN_POINT('Origin',(-4.505,3.4,72.85));
#47466=CARTESIAN_POINT('',(-4.505,3.4,72.85));
#47467=CARTESIAN_POINT('',(-4.505,-3.4,72.85));
#47468=CARTESIAN_POINT('',(-4.505,-0.3,72.85));
#47469=CARTESIAN_POINT('',(-4.655,3.4,72.85));
#47470=CARTESIAN_POINT('',(-4.505,3.4,72.85));
#47471=CARTESIAN_POINT('',(-4.655,-3.4,72.85));
#47472=CARTESIAN_POINT('',(-4.655,-3.4,72.85));
#47473=CARTESIAN_POINT('',(-4.505,-3.4,72.85));
#47474=CARTESIAN_POINT('Origin',(-4.505,3.4,73.15));
#47475=CARTESIAN_POINT('',(-4.505,3.4,73.15));
#47476=CARTESIAN_POINT('',(-4.505,3.4,69.325));
#47477=CARTESIAN_POINT('',(-4.655,3.4,73.15));
#47478=CARTESIAN_POINT('',(-4.505,3.4,73.15));
#47479=CARTESIAN_POINT('',(-4.655,3.4,72.85));
#47480=CARTESIAN_POINT('Origin',(-4.505,-3.4,73.15));
#47481=CARTESIAN_POINT('',(-4.505,-3.4,73.15));
#47482=CARTESIAN_POINT('',(-4.505,-3.7,73.15));
#47483=CARTESIAN_POINT('',(-4.655,-3.4,73.15));
#47484=CARTESIAN_POINT('',(-4.505,-3.4,73.15));
#47485=CARTESIAN_POINT('',(-4.655,3.4,73.15));
#47486=CARTESIAN_POINT('Origin',(-4.505,-3.4,72.85));
#47487=CARTESIAN_POINT('',(-4.505,-3.4,69.175));
#47488=CARTESIAN_POINT('',(-4.655,-3.4,73.15));
#47489=CARTESIAN_POINT('Origin',(-4.655,0.,73.));
#47490=CARTESIAN_POINT('Origin',(-5.895,-4.,76.4));
#47491=CARTESIAN_POINT('',(-5.995,-3.9,76.4));
#47492=CARTESIAN_POINT('',(-5.895,-3.9,76.5));
#47493=CARTESIAN_POINT('',(-5.995,-3.9,76.4));
#47494=CARTESIAN_POINT('',(-5.895,-4.,76.4));
#47495=CARTESIAN_POINT('',(-5.895,-4.,76.4));
#47496=CARTESIAN_POINT('',(-5.895,-3.9,76.5));
#47497=CARTESIAN_POINT('Origin',(-4.505,-3.9,76.4));
#47498=CARTESIAN_POINT('',(-4.605,-4.,76.4));
#47499=CARTESIAN_POINT('',(-4.605,-3.9,76.5));
#47500=CARTESIAN_POINT('',(-4.605,-4.,76.4));
#47501=CARTESIAN_POINT('',(-4.505,-3.9,76.4));
#47502=CARTESIAN_POINT('',(-4.505,-3.9,76.4));
#47503=CARTESIAN_POINT('',(-4.605,-3.9,76.5));
#47504=CARTESIAN_POINT('Origin',(-5.895,-3.9,65.5));
#47505=CARTESIAN_POINT('',(-5.995,-3.9,65.6));
#47506=CARTESIAN_POINT('',(-5.895,-4.,65.6));
#47507=CARTESIAN_POINT('',(-5.995,-3.9,65.6));
#47508=CARTESIAN_POINT('',(-5.895,-3.9,65.5));
#47509=CARTESIAN_POINT('',(-5.895,-3.9,65.5));
#47510=CARTESIAN_POINT('',(-5.895,-4.,65.6));
#47511=CARTESIAN_POINT('Origin',(-5.995,3.9,76.4));
#47512=CARTESIAN_POINT('',(-5.895,4.,76.4));
#47513=CARTESIAN_POINT('',(-5.895,3.9,76.5));
#47514=CARTESIAN_POINT('',(-5.895,4.,76.4));
#47515=CARTESIAN_POINT('',(-5.995,3.9,76.4));
#47516=CARTESIAN_POINT('',(-5.995,3.9,76.4));
#47517=CARTESIAN_POINT('',(-5.895,3.9,76.5));
#47518=CARTESIAN_POINT('Origin',(-4.605,-3.9,65.5));
#47519=CARTESIAN_POINT('',(-4.605,-4.,65.6));
#47520=CARTESIAN_POINT('',(-4.505,-3.9,65.6));
#47521=CARTESIAN_POINT('',(-4.605,-4.,65.6));
#47522=CARTESIAN_POINT('',(-4.605,-3.9,65.5));
#47523=CARTESIAN_POINT('',(-4.605,-3.9,65.5));
#47524=CARTESIAN_POINT('',(-4.505,-3.9,65.6));
#47525=CARTESIAN_POINT('Origin',(-5.6225,-3.95,65.55));
#47526=CARTESIAN_POINT('',(-5.6225,-4.,65.6));
#47527=CARTESIAN_POINT('',(-5.6225,-3.9,65.5));
#47528=CARTESIAN_POINT('Origin',(-4.605,4.,76.4));
#47529=CARTESIAN_POINT('',(-4.505,3.9,76.4));
#47530=CARTESIAN_POINT('',(-4.605,3.9,76.5));
#47531=CARTESIAN_POINT('',(-4.505,3.9,76.4));
#47532=CARTESIAN_POINT('',(-4.605,4.,76.4));
#47533=CARTESIAN_POINT('',(-4.605,4.,76.4));
#47534=CARTESIAN_POINT('',(-4.605,3.9,76.5));
#47535=CARTESIAN_POINT('Origin',(-5.995,3.9,65.6));
#47536=CARTESIAN_POINT('',(-5.895,3.9,65.5));
#47537=CARTESIAN_POINT('',(-5.895,4.,65.6));
#47538=CARTESIAN_POINT('',(-5.895,3.9,65.5));
#47539=CARTESIAN_POINT('',(-5.995,3.9,65.6));
#47540=CARTESIAN_POINT('',(-5.995,3.9,65.6));
#47541=CARTESIAN_POINT('',(-5.895,4.,65.6));
#47542=CARTESIAN_POINT('Origin',(-5.945,2.,65.55));
#47543=CARTESIAN_POINT('',(-5.995,2.,65.6));
#47544=CARTESIAN_POINT('',(-5.895,2.,65.5));
#47545=CARTESIAN_POINT('Origin',(-5.945,3.95,65.5));
#47546=CARTESIAN_POINT('',(-5.895,4.,65.5));
#47547=CARTESIAN_POINT('',(-5.995,3.9,65.5));
#47548=CARTESIAN_POINT('Origin',(-4.605,3.9,65.5));
#47549=CARTESIAN_POINT('',(-4.505,3.9,65.6));
#47550=CARTESIAN_POINT('',(-4.605,4.,65.6));
#47551=CARTESIAN_POINT('',(-4.505,3.9,65.6));
#47552=CARTESIAN_POINT('',(-4.605,3.9,65.5));
#47553=CARTESIAN_POINT('',(-4.605,3.9,65.5));
#47554=CARTESIAN_POINT('',(-4.605,4.,65.6));
#47555=CARTESIAN_POINT('Origin',(-4.555,-2.,65.55));
#47556=CARTESIAN_POINT('',(-4.505,-2.,65.6));
#47557=CARTESIAN_POINT('',(-4.605,-2.,65.5));
#47558=CARTESIAN_POINT('Origin',(-4.8775,3.95,65.55));
#47559=CARTESIAN_POINT('',(-4.8775,4.,65.6));
#47560=CARTESIAN_POINT('',(-4.8775,3.9,65.5));
#47561=CARTESIAN_POINT('Origin',(-4.555,3.95,65.5));
#47562=CARTESIAN_POINT('',(-4.505,3.9,65.5));
#47563=CARTESIAN_POINT('',(-4.605,4.,65.5));
#47564=CARTESIAN_POINT('Origin',(-4.8775,3.95,76.45));
#47565=CARTESIAN_POINT('',(-4.8775,3.9,76.5));
#47566=CARTESIAN_POINT('',(-4.8775,4.,76.4));
#47567=CARTESIAN_POINT('Origin',(-4.555,-2.,76.45));
#47568=CARTESIAN_POINT('',(-4.605,-2.,76.5));
#47569=CARTESIAN_POINT('',(-4.505,-2.,76.4));
#47570=CARTESIAN_POINT('Origin',(-4.555,-3.95,65.5));
#47571=CARTESIAN_POINT('',(-4.605,-4.,65.5));
#47572=CARTESIAN_POINT('',(-4.505,-3.9,65.5));
#47573=CARTESIAN_POINT('Origin',(-5.945,2.,76.45));
#47574=CARTESIAN_POINT('',(-5.895,2.,76.5));
#47575=CARTESIAN_POINT('',(-5.995,2.,76.4));
#47576=CARTESIAN_POINT('Origin',(-5.945,-3.95,65.5));
#47577=CARTESIAN_POINT('',(-5.995,-3.9,65.5));
#47578=CARTESIAN_POINT('',(-5.895,-4.,65.5));
#47579=CARTESIAN_POINT('Origin',(-5.6225,-3.95,76.45));
#47580=CARTESIAN_POINT('',(-5.6225,-3.9,76.5));
#47581=CARTESIAN_POINT('',(-5.6225,-4.,76.4));
#47582=CARTESIAN_POINT('Origin',(-5.995,-4.,65.5));
#47583=CARTESIAN_POINT('Origin',(-5.25,0.,65.5));
#47584=CARTESIAN_POINT('Origin',(-5.995,4.,65.5));
#47585=CARTESIAN_POINT('Origin',(-4.505,4.,65.5));
#47586=CARTESIAN_POINT('Origin',(-4.505,-4.,65.5));
#47587=CARTESIAN_POINT('Origin',(-5.25,0.,76.5));
#70731=UNCERTAINTY_MEASURE_WITH_UNIT(LENGTH_MEASURE(0.001),#70758,
'DISTANCE_ACCURACY_VALUE',
'Maximum model space distance between geometric entities at asserted c
onnectivities');
#70740=UNCERTAINTY_MEASURE_WITH_UNIT(LENGTH_MEASURE(0.001),#70758,
'DISTANCE_ACCURACY_VALUE',
'Maximum model space distance between geometric entities at asserted c
onnectivities');
#70748=(
GEOMETRIC_REPRESENTATION_CONTEXT(3)
GLOBAL_UNCERTAINTY_ASSIGNED_CONTEXT((#70731))
GLOBAL_UNIT_ASSIGNED_CONTEXT((#70758,#70760,#70761))
REPRESENTATION_CONTEXT('','3D')
);
#70757=(
GEOMETRIC_REPRESENTATION_CONTEXT(3)
GLOBAL_UNCERTAINTY_ASSIGNED_CONTEXT((#70740))
GLOBAL_UNIT_ASSIGNED_CONTEXT((#70758,#70760,#70761))
REPRESENTATION_CONTEXT('','3D')
);
#70758=(
LENGTH_UNIT()
NAMED_UNIT(*)
SI_UNIT(.CENTI.,.METRE.)
);
#70760=(
NAMED_UNIT(*)
PLANE_ANGLE_UNIT()
SI_UNIT($,.RADIAN.)
);
#70761=(
NAMED_UNIT(*)
SI_UNIT($,.STERADIAN.)
SOLID_ANGLE_UNIT()
);
#70769=SHAPE_DEFINITION_REPRESENTATION(#70785,#70824);
#70785=PRODUCT_DEFINITION_SHAPE('',$,#70841);
#70824=SHAPE_REPRESENTATION('',(#27510),#70748);
#70833=PRODUCT_DEFINITION_CONTEXT('part definition',#70883,'design');
#70841=PRODUCT_DEFINITION('2026-10-19-02-55-37-006',
'10_Ram_Guide_Gib_Wear_Plate_110x80x14.9',#70857,#70833);
#70857=PRODUCT_DEFINITION_FORMATION('',$,#70892);
#70883=APPLICATION_CONTEXT(
'Core Data for Automotive Mechanical Design Process');
#70884=PRODUCT_CONTEXT('part definition',#70883,'mechanical');
#70892=PRODUCT('2026-10-19-02-55-37-006',
'10_Ram_Guide_Gib_Wear_Plate_110x80x14.9',$,(#70884));
#71034=COLOUR_RGB('Sky Blue',0.24,0.69,0.87);
#71035=FILL_AREA_STYLE_COLOUR('',#71034);
#71036=FILL_AREA_STYLE('',(#71035));
#71037=SURFACE_STYLE_FILL_AREA(#71036);
#71038=SURFACE_SIDE_STYLE('',(#71037));
#71039=SURFACE_STYLE_USAGE(.BOTH.,#71038);
#71040=PRESENTATION_STYLE_ASSIGNMENT((#71039));
ENDSEC;
END-ISO-10303-21;
